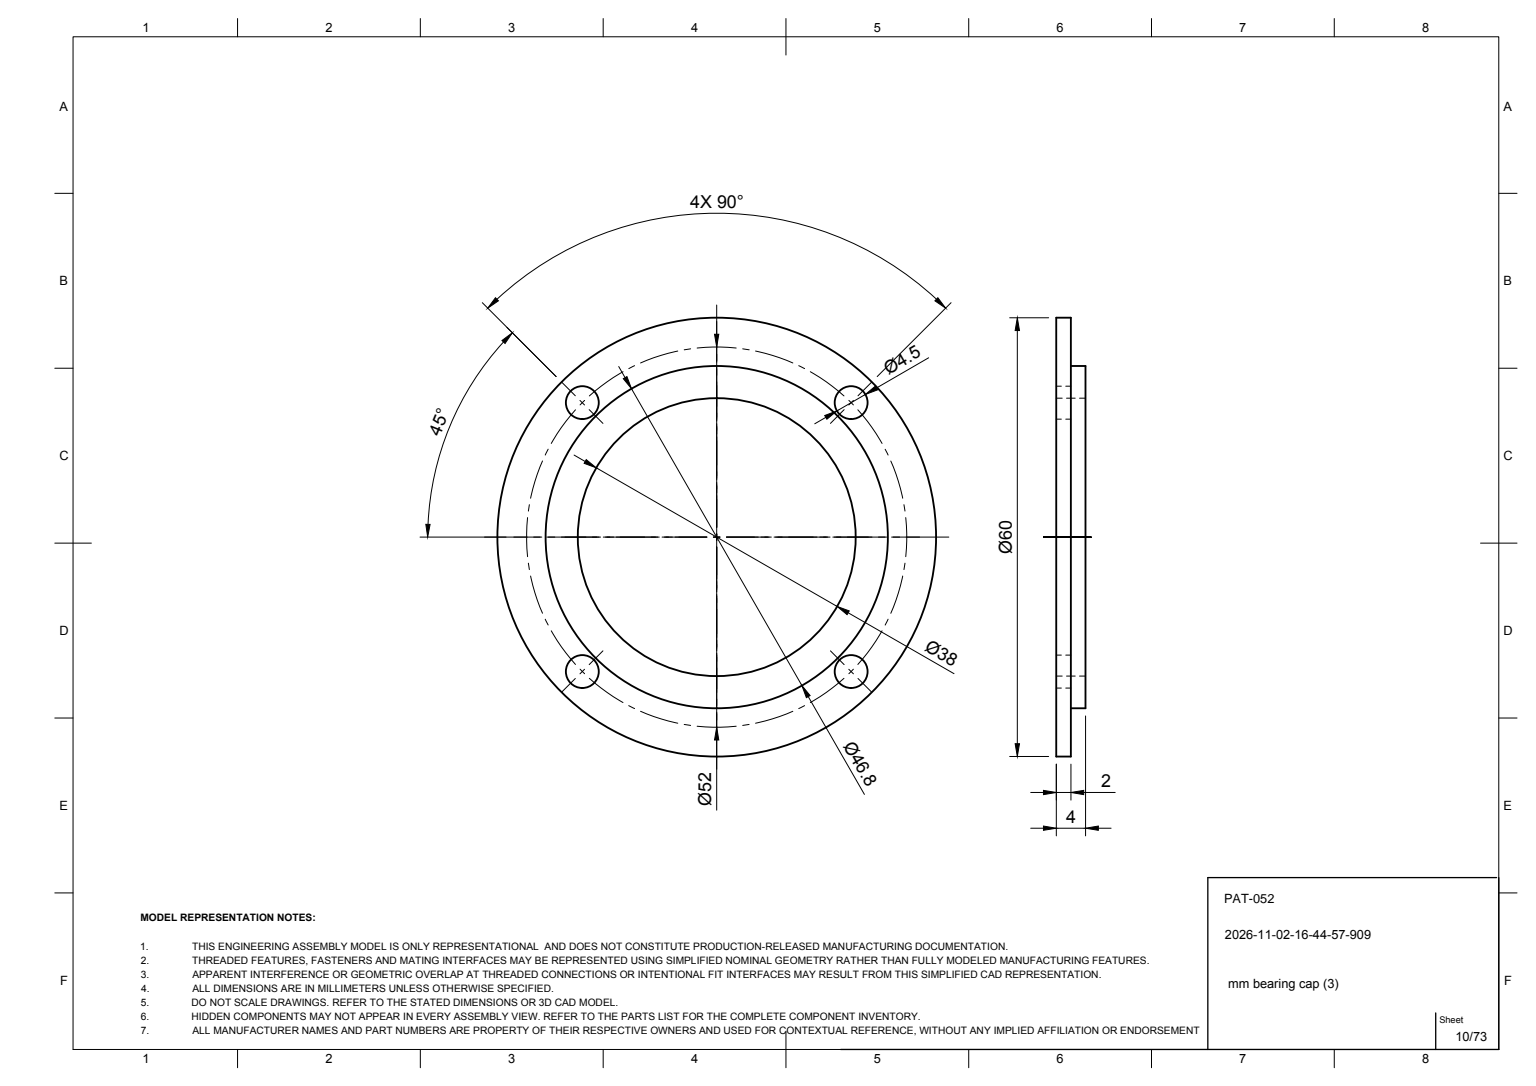
ISO-10303-21;
HEADER;
/* Generated by software containing ST-Developer
 * from STEP Tools, Inc. (www.steptools.com) 
 */

FILE_DESCRIPTION(
/* description */ ('Hand-crank gear train demonstrator'),
/* implementation_level */ '2;1');

FILE_NAME(
/* name */ 'mm bearing cap (3).step',
/* time_stamp */ '2026-10-28T03:22:13-07:00',
/* author */ (''),
/* organization */ (''),
/* preprocessor_version */ 'ST-DEVELOPER v20.2',
/* originating_system */ 'Autodesk Translation Framework v15.17.0.0',
/* authorisation */ '');

FILE_SCHEMA (('AUTOMOTIVE_DESIGN { 1 0 10303 214 3 1 1 }'));
ENDSEC;

DATA;
#10=MECHANICAL_DESIGN_GEOMETRIC_PRESENTATION_REPRESENTATION('',(#1194),#62758);
#1066=SHAPE_REPRESENTATION_RELATIONSHIP('SRR','None',#63038,#1130);
#1130=ADVANCED_BREP_SHAPE_REPRESENTATION('',(#1273),#62692);
#1194=STYLED_ITEM('',(#63462),#1273);
#1273=MANIFOLD_SOLID_BREP('Body1',#16374);
#1431=FACE_BOUND('',#3226,.T.);
#1432=FACE_BOUND('',#3230,.T.);
#1433=FACE_BOUND('',#3231,.T.);
#1434=FACE_BOUND('',#3232,.T.);
#1435=FACE_BOUND('',#3233,.T.);
#1436=FACE_BOUND('',#3234,.T.);
#1437=FACE_BOUND('',#3236,.T.);
#1438=FACE_BOUND('',#3237,.T.);
#1439=FACE_BOUND('',#3238,.T.);
#1440=FACE_BOUND('',#3239,.T.);
#1441=FACE_BOUND('',#3240,.T.);
#1656=PLANE('',#17351);
#1657=PLANE('',#17358);
#1658=PLANE('',#17359);
#2195=FACE_OUTER_BOUND('',#3220,.T.);
#2196=FACE_OUTER_BOUND('',#3221,.T.);
#2197=FACE_OUTER_BOUND('',#3222,.T.);
#2198=FACE_OUTER_BOUND('',#3223,.T.);
#2199=FACE_OUTER_BOUND('',#3224,.T.);
#2200=FACE_OUTER_BOUND('',#3225,.T.);
#2201=FACE_OUTER_BOUND('',#3227,.T.);
#2202=FACE_OUTER_BOUND('',#3228,.T.);
#2203=FACE_OUTER_BOUND('',#3229,.T.);
#2204=FACE_OUTER_BOUND('',#3235,.T.);
#3220=EDGE_LOOP('',(#11189,#11190,#11191,#11192));
#3221=EDGE_LOOP('',(#11193,#11194,#11195,#11196));
#3222=EDGE_LOOP('',(#11197,#11198,#11199,#11200));
#3223=EDGE_LOOP('',(#11201,#11202,#11203,#11204));
#3224=EDGE_LOOP('',(#11205,#11206,#11207,#11208));
#3225=EDGE_LOOP('',(#11209));
#3226=EDGE_LOOP('',(#11210));
#3227=EDGE_LOOP('',(#11211,#11212,#11213,#11214));
#3228=EDGE_LOOP('',(#11215,#11216,#11217,#11218));
#3229=EDGE_LOOP('',(#11219));
#3230=EDGE_LOOP('',(#11220));
#3231=EDGE_LOOP('',(#11221));
#3232=EDGE_LOOP('',(#11222));
#3233=EDGE_LOOP('',(#11223));
#3234=EDGE_LOOP('',(#11224));
#3235=EDGE_LOOP('',(#11225));
#3236=EDGE_LOOP('',(#11226));
#3237=EDGE_LOOP('',(#11227));
#3238=EDGE_LOOP('',(#11228));
#3239=EDGE_LOOP('',(#11229));
#3240=EDGE_LOOP('',(#11230));
#4365=LINE('',#23688,#5497);
#4366=LINE('',#23694,#5498);
#4367=LINE('',#23700,#5499);
#4368=LINE('',#23706,#5500);
#4369=LINE('',#23712,#5501);
#4370=LINE('',#23720,#5502);
#4371=LINE('',#23725,#5503);
#5497=VECTOR('',#19270,0.225);
#5498=VECTOR('',#19277,0.225);
#5499=VECTOR('',#19284,0.225000000000001);
#5500=VECTOR('',#19291,0.225000000000001);
#5501=VECTOR('',#19298,2.34);
#5502=VECTOR('',#19309,1.9);
#5503=VECTOR('',#19314,3.);
#6648=CIRCLE('',#17337,0.225);
#6649=CIRCLE('',#17338,0.225);
#6650=CIRCLE('',#17340,0.225);
#6651=CIRCLE('',#17341,0.225);
#6652=CIRCLE('',#17343,0.225000000000001);
#6653=CIRCLE('',#17344,0.225000000000001);
#6654=CIRCLE('',#17346,0.225000000000001);
#6655=CIRCLE('',#17347,0.225000000000001);
#6656=CIRCLE('',#17349,2.34);
#6657=CIRCLE('',#17350,2.34);
#6658=CIRCLE('',#17352,1.9);
#6659=CIRCLE('',#17354,1.9);
#6660=CIRCLE('',#17356,3.);
#6661=CIRCLE('',#17357,3.);
#7330=VERTEX_POINT('',#23685);
#7331=VERTEX_POINT('',#23687);
#7332=VERTEX_POINT('',#23691);
#7333=VERTEX_POINT('',#23693);
#7334=VERTEX_POINT('',#23697);
#7335=VERTEX_POINT('',#23699);
#7336=VERTEX_POINT('',#23703);
#7337=VERTEX_POINT('',#23705);
#7338=VERTEX_POINT('',#23709);
#7339=VERTEX_POINT('',#23711);
#7340=VERTEX_POINT('',#23715);
#7341=VERTEX_POINT('',#23718);
#7342=VERTEX_POINT('',#23722);
#7343=VERTEX_POINT('',#23724);
#8846=EDGE_CURVE('',#7330,#7330,#6648,.T.);
#8847=EDGE_CURVE('',#7330,#7331,#4365,.T.);
#8848=EDGE_CURVE('',#7331,#7331,#6649,.T.);
#8849=EDGE_CURVE('',#7332,#7332,#6650,.T.);
#8850=EDGE_CURVE('',#7332,#7333,#4366,.T.);
#8851=EDGE_CURVE('',#7333,#7333,#6651,.T.);
#8852=EDGE_CURVE('',#7334,#7334,#6652,.T.);
#8853=EDGE_CURVE('',#7334,#7335,#4367,.T.);
#8854=EDGE_CURVE('',#7335,#7335,#6653,.T.);
#8855=EDGE_CURVE('',#7336,#7336,#6654,.T.);
#8856=EDGE_CURVE('',#7336,#7337,#4368,.T.);
#8857=EDGE_CURVE('',#7337,#7337,#6655,.T.);
#8858=EDGE_CURVE('',#7338,#7338,#6656,.T.);
#8859=EDGE_CURVE('',#7338,#7339,#4369,.T.);
#8860=EDGE_CURVE('',#7339,#7339,#6657,.T.);
#8861=EDGE_CURVE('',#7340,#7340,#6658,.T.);
#8862=EDGE_CURVE('',#7341,#7341,#6659,.T.);
#8863=EDGE_CURVE('',#7341,#7340,#4370,.T.);
#8864=EDGE_CURVE('',#7342,#7342,#6660,.T.);
#8865=EDGE_CURVE('',#7342,#7343,#4371,.T.);
#8866=EDGE_CURVE('',#7343,#7343,#6661,.T.);
#11189=ORIENTED_EDGE('',*,*,#8846,.F.);
#11190=ORIENTED_EDGE('',*,*,#8847,.T.);
#11191=ORIENTED_EDGE('',*,*,#8848,.F.);
#11192=ORIENTED_EDGE('',*,*,#8847,.F.);
#11193=ORIENTED_EDGE('',*,*,#8849,.F.);
#11194=ORIENTED_EDGE('',*,*,#8850,.T.);
#11195=ORIENTED_EDGE('',*,*,#8851,.F.);
#11196=ORIENTED_EDGE('',*,*,#8850,.F.);
#11197=ORIENTED_EDGE('',*,*,#8852,.F.);
#11198=ORIENTED_EDGE('',*,*,#8853,.T.);
#11199=ORIENTED_EDGE('',*,*,#8854,.F.);
#11200=ORIENTED_EDGE('',*,*,#8853,.F.);
#11201=ORIENTED_EDGE('',*,*,#8855,.F.);
#11202=ORIENTED_EDGE('',*,*,#8856,.T.);
#11203=ORIENTED_EDGE('',*,*,#8857,.F.);
#11204=ORIENTED_EDGE('',*,*,#8856,.F.);
#11205=ORIENTED_EDGE('',*,*,#8858,.F.);
#11206=ORIENTED_EDGE('',*,*,#8859,.T.);
#11207=ORIENTED_EDGE('',*,*,#8860,.T.);
#11208=ORIENTED_EDGE('',*,*,#8859,.F.);
#11209=ORIENTED_EDGE('',*,*,#8860,.F.);
#11210=ORIENTED_EDGE('',*,*,#8861,.F.);
#11211=ORIENTED_EDGE('',*,*,#8862,.F.);
#11212=ORIENTED_EDGE('',*,*,#8863,.T.);
#11213=ORIENTED_EDGE('',*,*,#8861,.T.);
#11214=ORIENTED_EDGE('',*,*,#8863,.F.);
#11215=ORIENTED_EDGE('',*,*,#8864,.F.);
#11216=ORIENTED_EDGE('',*,*,#8865,.T.);
#11217=ORIENTED_EDGE('',*,*,#8866,.T.);
#11218=ORIENTED_EDGE('',*,*,#8865,.F.);
#11219=ORIENTED_EDGE('',*,*,#8864,.T.);
#11220=ORIENTED_EDGE('',*,*,#8862,.T.);
#11221=ORIENTED_EDGE('',*,*,#8857,.T.);
#11222=ORIENTED_EDGE('',*,*,#8854,.T.);
#11223=ORIENTED_EDGE('',*,*,#8851,.T.);
#11224=ORIENTED_EDGE('',*,*,#8848,.T.);
#11225=ORIENTED_EDGE('',*,*,#8866,.F.);
#11226=ORIENTED_EDGE('',*,*,#8858,.T.);
#11227=ORIENTED_EDGE('',*,*,#8855,.T.);
#11228=ORIENTED_EDGE('',*,*,#8852,.T.);
#11229=ORIENTED_EDGE('',*,*,#8849,.T.);
#11230=ORIENTED_EDGE('',*,*,#8846,.T.);
#15216=CYLINDRICAL_SURFACE('',#17336,0.225);
#15217=CYLINDRICAL_SURFACE('',#17339,0.225);
#15218=CYLINDRICAL_SURFACE('',#17342,0.225000000000001);
#15219=CYLINDRICAL_SURFACE('',#17345,0.225000000000001);
#15220=CYLINDRICAL_SURFACE('',#17348,2.34);
#15221=CYLINDRICAL_SURFACE('',#17353,1.9);
#15222=CYLINDRICAL_SURFACE('',#17355,3.);
#15505=ADVANCED_FACE('',(#2195),#15216,.F.);
#15506=ADVANCED_FACE('',(#2196),#15217,.F.);
#15507=ADVANCED_FACE('',(#2197),#15218,.F.);
#15508=ADVANCED_FACE('',(#2198),#15219,.F.);
#15509=ADVANCED_FACE('',(#2199),#15220,.T.);
#15510=ADVANCED_FACE('',(#2200,#1431),#1656,.F.);
#15511=ADVANCED_FACE('',(#2201),#15221,.F.);
#15512=ADVANCED_FACE('',(#2202),#15222,.T.);
#15513=ADVANCED_FACE('',(#2203,#1432,#1433,#1434,#1435,#1436),#1657,.T.);
#15514=ADVANCED_FACE('',(#2204,#1437,#1438,#1439,#1440,#1441),#1658,.F.);
#16374=CLOSED_SHELL('',(#15505,#15506,#15507,#15508,#15509,#15510,#15511,
#15512,#15513,#15514));
#17335=AXIS2_PLACEMENT_3D('',#23683,#19264,#19265);
#17336=AXIS2_PLACEMENT_3D('',#23684,#19266,#19267);
#17337=AXIS2_PLACEMENT_3D('',#23686,#19268,#19269);
#17338=AXIS2_PLACEMENT_3D('',#23689,#19271,#19272);
#17339=AXIS2_PLACEMENT_3D('',#23690,#19273,#19274);
#17340=AXIS2_PLACEMENT_3D('',#23692,#19275,#19276);
#17341=AXIS2_PLACEMENT_3D('',#23695,#19278,#19279);
#17342=AXIS2_PLACEMENT_3D('',#23696,#19280,#19281);
#17343=AXIS2_PLACEMENT_3D('',#23698,#19282,#19283);
#17344=AXIS2_PLACEMENT_3D('',#23701,#19285,#19286);
#17345=AXIS2_PLACEMENT_3D('',#23702,#19287,#19288);
#17346=AXIS2_PLACEMENT_3D('',#23704,#19289,#19290);
#17347=AXIS2_PLACEMENT_3D('',#23707,#19292,#19293);
#17348=AXIS2_PLACEMENT_3D('',#23708,#19294,#19295);
#17349=AXIS2_PLACEMENT_3D('',#23710,#19296,#19297);
#17350=AXIS2_PLACEMENT_3D('',#23713,#19299,#19300);
#17351=AXIS2_PLACEMENT_3D('',#23714,#19301,#19302);
#17352=AXIS2_PLACEMENT_3D('',#23716,#19303,#19304);
#17353=AXIS2_PLACEMENT_3D('',#23717,#19305,#19306);
#17354=AXIS2_PLACEMENT_3D('',#23719,#19307,#19308);
#17355=AXIS2_PLACEMENT_3D('',#23721,#19310,#19311);
#17356=AXIS2_PLACEMENT_3D('',#23723,#19312,#19313);
#17357=AXIS2_PLACEMENT_3D('',#23726,#19315,#19316);
#17358=AXIS2_PLACEMENT_3D('',#23727,#19317,#19318);
#17359=AXIS2_PLACEMENT_3D('',#23728,#19319,#19320);
#19264=DIRECTION('axis',(0.,0.,1.));
#19265=DIRECTION('refdir',(1.,0.,0.));
#19266=DIRECTION('center_axis',(0.,1.,0.));
#19267=DIRECTION('ref_axis',(1.,0.,0.));
#19268=DIRECTION('center_axis',(0.,1.,0.));
#19269=DIRECTION('ref_axis',(1.,0.,0.));
#19270=DIRECTION('',(0.,1.,0.));
#19271=DIRECTION('center_axis',(0.,-1.,0.));
#19272=DIRECTION('ref_axis',(1.,0.,0.));
#19273=DIRECTION('center_axis',(0.,1.,0.));
#19274=DIRECTION('ref_axis',(1.,0.,0.));
#19275=DIRECTION('center_axis',(0.,1.,0.));
#19276=DIRECTION('ref_axis',(1.,0.,0.));
#19277=DIRECTION('',(0.,1.,0.));
#19278=DIRECTION('center_axis',(0.,-1.,0.));
#19279=DIRECTION('ref_axis',(1.,0.,0.));
#19280=DIRECTION('center_axis',(0.,1.,0.));
#19281=DIRECTION('ref_axis',(1.,0.,0.));
#19282=DIRECTION('center_axis',(0.,1.,0.));
#19283=DIRECTION('ref_axis',(1.,0.,0.));
#19284=DIRECTION('',(0.,1.,0.));
#19285=DIRECTION('center_axis',(0.,-1.,0.));
#19286=DIRECTION('ref_axis',(1.,0.,0.));
#19287=DIRECTION('center_axis',(0.,1.,0.));
#19288=DIRECTION('ref_axis',(1.,0.,0.));
#19289=DIRECTION('center_axis',(0.,1.,0.));
#19290=DIRECTION('ref_axis',(1.,0.,0.));
#19291=DIRECTION('',(0.,1.,0.));
#19292=DIRECTION('center_axis',(0.,-1.,0.));
#19293=DIRECTION('ref_axis',(1.,0.,0.));
#19294=DIRECTION('center_axis',(0.,1.,0.));
#19295=DIRECTION('ref_axis',(1.,0.,0.));
#19296=DIRECTION('center_axis',(0.,1.,0.));
#19297=DIRECTION('ref_axis',(1.,0.,0.));
#19298=DIRECTION('',(0.,-1.,0.));
#19299=DIRECTION('center_axis',(0.,1.,0.));
#19300=DIRECTION('ref_axis',(1.,0.,0.));
#19301=DIRECTION('center_axis',(0.,1.,0.));
#19302=DIRECTION('ref_axis',(1.,0.,0.));
#19303=DIRECTION('center_axis',(0.,-1.,0.));
#19304=DIRECTION('ref_axis',(1.,0.,0.));
#19305=DIRECTION('center_axis',(0.,1.,0.));
#19306=DIRECTION('ref_axis',(1.,0.,0.));
#19307=DIRECTION('center_axis',(0.,-1.,0.));
#19308=DIRECTION('ref_axis',(1.,0.,0.));
#19309=DIRECTION('',(0.,-1.,0.));
#19310=DIRECTION('center_axis',(0.,1.,0.));
#19311=DIRECTION('ref_axis',(1.,0.,0.));
#19312=DIRECTION('center_axis',(0.,1.,0.));
#19313=DIRECTION('ref_axis',(1.,0.,0.));
#19314=DIRECTION('',(0.,-1.,0.));
#19315=DIRECTION('center_axis',(0.,1.,0.));
#19316=DIRECTION('ref_axis',(1.,0.,0.));
#19317=DIRECTION('center_axis',(0.,1.,0.));
#19318=DIRECTION('ref_axis',(1.,0.,0.));
#19319=DIRECTION('center_axis',(0.,1.,0.));
#19320=DIRECTION('ref_axis',(1.,0.,0.));
#23683=CARTESIAN_POINT('',(0.,0.,0.));
#23684=CARTESIAN_POINT('Origin',(4.16152236891498,-0.7,7.16152236891498));
#23685=CARTESIAN_POINT('',(3.93652236891498,-0.6,7.16152236891498));
#23686=CARTESIAN_POINT('Origin',(4.16152236891498,-0.6,7.16152236891498));
#23687=CARTESIAN_POINT('',(3.93652236891498,-0.4,7.16152236891498));
#23688=CARTESIAN_POINT('',(3.93652236891498,-0.7,7.16152236891498));
#23689=CARTESIAN_POINT('Origin',(4.16152236891498,-0.4,7.16152236891498));
#23690=CARTESIAN_POINT('Origin',(4.16152236891498,-0.7,10.838477631085));
#23691=CARTESIAN_POINT('',(3.93652236891498,-0.6,10.838477631085));
#23692=CARTESIAN_POINT('Origin',(4.16152236891498,-0.6,10.838477631085));
#23693=CARTESIAN_POINT('',(3.93652236891498,-0.4,10.838477631085));
#23694=CARTESIAN_POINT('',(3.93652236891498,-0.7,10.838477631085));
#23695=CARTESIAN_POINT('Origin',(4.16152236891498,-0.4,10.838477631085));
#23696=CARTESIAN_POINT('Origin',(7.83847763108502,-0.7,10.838477631085));
#23697=CARTESIAN_POINT('',(7.61347763108502,-0.6,10.838477631085));
#23698=CARTESIAN_POINT('Origin',(7.83847763108502,-0.6,10.838477631085));
#23699=CARTESIAN_POINT('',(7.61347763108502,-0.4,10.838477631085));
#23700=CARTESIAN_POINT('',(7.61347763108502,-0.7,10.838477631085));
#23701=CARTESIAN_POINT('Origin',(7.83847763108502,-0.4,10.838477631085));
#23702=CARTESIAN_POINT('Origin',(7.83847763108502,-0.7,7.16152236891498));
#23703=CARTESIAN_POINT('',(7.61347763108502,-0.6,7.16152236891498));
#23704=CARTESIAN_POINT('Origin',(7.83847763108502,-0.6,7.16152236891498));
#23705=CARTESIAN_POINT('',(7.61347763108502,-0.4,7.16152236891498));
#23706=CARTESIAN_POINT('',(7.61347763108502,-0.7,7.16152236891498));
#23707=CARTESIAN_POINT('Origin',(7.83847763108502,-0.4,7.16152236891498));
#23708=CARTESIAN_POINT('Origin',(6.,-0.8,9.));
#23709=CARTESIAN_POINT('',(3.66,-0.6,9.));
#23710=CARTESIAN_POINT('Origin',(6.,-0.6,9.));
#23711=CARTESIAN_POINT('',(3.66,-0.8,9.));
#23712=CARTESIAN_POINT('',(3.66,-0.8,9.));
#23713=CARTESIAN_POINT('Origin',(6.,-0.8,9.));
#23714=CARTESIAN_POINT('Origin',(6.,-0.8,9.));
#23715=CARTESIAN_POINT('',(4.1,-0.8,9.));
#23716=CARTESIAN_POINT('Origin',(6.,-0.8,9.));
#23717=CARTESIAN_POINT('Origin',(6.,-0.6,9.));
#23718=CARTESIAN_POINT('',(4.1,-0.4,9.));
#23719=CARTESIAN_POINT('Origin',(6.,-0.4,9.));
#23720=CARTESIAN_POINT('',(4.1,-0.6,9.));
#23721=CARTESIAN_POINT('Origin',(6.,-0.6,9.));
#23722=CARTESIAN_POINT('',(3.,-0.4,9.));
#23723=CARTESIAN_POINT('Origin',(6.,-0.4,9.));
#23724=CARTESIAN_POINT('',(3.,-0.6,9.));
#23725=CARTESIAN_POINT('',(3.,-0.6,9.));
#23726=CARTESIAN_POINT('Origin',(6.,-0.6,9.));
#23727=CARTESIAN_POINT('Origin',(6.,-0.4,9.));
#23728=CARTESIAN_POINT('Origin',(6.,-0.6,9.));
#62618=UNCERTAINTY_MEASURE_WITH_UNIT(LENGTH_MEASURE(0.001),#62759,
'DISTANCE_ACCURACY_VALUE',
'Maximum model space distance between geometric entities at asserted c
onnectivities');
#62684=UNCERTAINTY_MEASURE_WITH_UNIT(LENGTH_MEASURE(0.001),#62759,
'DISTANCE_ACCURACY_VALUE',
'Maximum model space distance between geometric entities at asserted c
onnectivities');
#62692=(
GEOMETRIC_REPRESENTATION_CONTEXT(3)
GLOBAL_UNCERTAINTY_ASSIGNED_CONTEXT((#62618))
GLOBAL_UNIT_ASSIGNED_CONTEXT((#62759,#62761,#62762))
REPRESENTATION_CONTEXT('','3D')
);
#62758=(
GEOMETRIC_REPRESENTATION_CONTEXT(3)
GLOBAL_UNCERTAINTY_ASSIGNED_CONTEXT((#62684))
GLOBAL_UNIT_ASSIGNED_CONTEXT((#62759,#62761,#62762))
REPRESENTATION_CONTEXT('','3D')
);
#62759=(
LENGTH_UNIT()
NAMED_UNIT(*)
SI_UNIT(.CENTI.,.METRE.)
);
#62761=(
NAMED_UNIT(*)
PLANE_ANGLE_UNIT()
SI_UNIT($,.RADIAN.)
);
#62762=(
NAMED_UNIT(*)
SI_UNIT($,.STERADIAN.)
SOLID_ANGLE_UNIT()
);
#62770=SHAPE_DEFINITION_REPRESENTATION(#62843,#63038);
#62843=PRODUCT_DEFINITION_SHAPE('',$,#63112);
#63038=SHAPE_REPRESENTATION('',(#17335),#62692);
#63104=PRODUCT_DEFINITION_CONTEXT('part definition',#63325,'design');
#63112=PRODUCT_DEFINITION('mm bearing cap (3)','mm bearing cap (3)',#63185,
#63104);
#63185=PRODUCT_DEFINITION_FORMATION('',$,#63334);
#63325=APPLICATION_CONTEXT(
'Core Data for Automotive Mechanical Design Process');
#63326=PRODUCT_CONTEXT('part definition',#63325,'mechanical');
#63334=PRODUCT('mm bearing cap (3)','mm bearing cap (3)','mm bearing cap (3)',
(#63326));
#63456=COLOUR_RGB('Grey',0.48,0.52,0.57);
#63457=FILL_AREA_STYLE_COLOUR('',#63456);
#63458=FILL_AREA_STYLE('',(#63457));
#63459=SURFACE_STYLE_FILL_AREA(#63458);
#63460=SURFACE_SIDE_STYLE('',(#63459));
#63461=SURFACE_STYLE_USAGE(.BOTH.,#63460);
#63462=PRESENTATION_STYLE_ASSIGNMENT((#63461));
ENDSEC;
END-ISO-10303-21;
